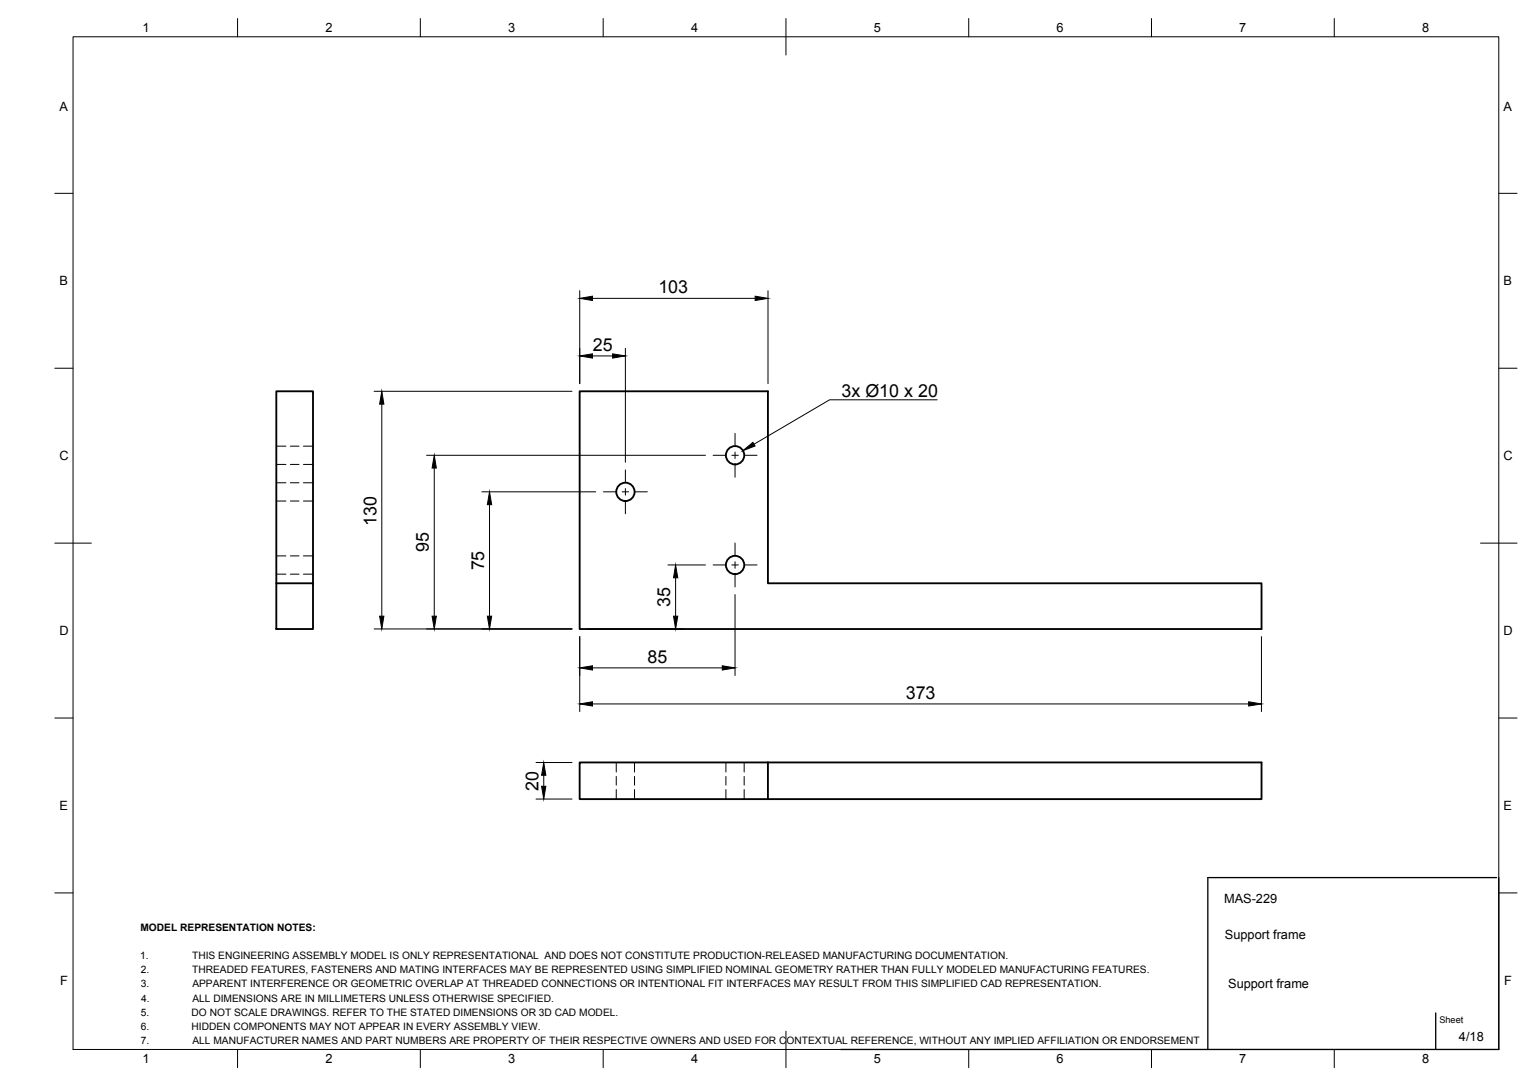
ISO-10303-21;
HEADER;
/* Generated by software containing ST-Developer
 * from STEP Tools, Inc. (www.steptools.com) 
 */

FILE_DESCRIPTION(
/* description */ ('Independently dimensioned six-bar single-leg walking-linkage demonstr
ator. Whole-mm20 crank,60 upper rocker,80/120 ternary coupler,120 lowe
r rocker,140 knee pitch and260 toe reach; ground pivots0/0,60/0,40/60.
 Seven native revolutes close both loops. Four reused native library f
amilies, fully retained shared pins and layered real spacer stacks, bo
nded rubber toe. Benchtop reference mechanism; no complete vehicle, lo
ad, gait stability, adhesive, weld, fit or life rating.'),
/* implementation_level */ '2;1');

FILE_NAME(
/* name */ 'Support frame.step',
/* time_stamp */ '2026-11-09T20:33:14-08:00',
/* author */ (''),
/* organization */ (''),
/* preprocessor_version */ 'ST-DEVELOPER v20.2',
/* originating_system */ 'Autodesk Translation Framework v15.17.0.0',
/* authorisation */ '');

FILE_SCHEMA (('AUTOMOTIVE_DESIGN { 1 0 10303 214 3 1 1 }'));
ENDSEC;

DATA;
#10=MECHANICAL_DESIGN_GEOMETRIC_PRESENTATION_REPRESENTATION('',(#256),#4048);
#220=SHAPE_REPRESENTATION_RELATIONSHIP('SRR','None',#4144,#238);
#238=ADVANCED_BREP_SHAPE_REPRESENTATION('',(#274),#4031);
#256=STYLED_ITEM('',(#4243),#274);
#274=MANIFOLD_SOLID_BREP('Body1',#2145);
#299=FACE_BOUND('',#569,.T.);
#300=FACE_BOUND('',#570,.T.);
#301=FACE_BOUND('',#571,.T.);
#302=FACE_BOUND('',#573,.T.);
#303=FACE_BOUND('',#574,.T.);
#304=FACE_BOUND('',#575,.T.);
#354=PLANE('',#2391);
#355=PLANE('',#2392);
#356=PLANE('',#2393);
#357=PLANE('',#2394);
#358=PLANE('',#2395);
#359=PLANE('',#2396);
#360=PLANE('',#2397);
#361=PLANE('',#2398);
#425=FACE_OUTER_BOUND('',#559,.T.);
#426=FACE_OUTER_BOUND('',#560,.T.);
#427=FACE_OUTER_BOUND('',#561,.T.);
#428=FACE_OUTER_BOUND('',#562,.T.);
#429=FACE_OUTER_BOUND('',#563,.T.);
#430=FACE_OUTER_BOUND('',#564,.T.);
#431=FACE_OUTER_BOUND('',#565,.T.);
#432=FACE_OUTER_BOUND('',#566,.T.);
#433=FACE_OUTER_BOUND('',#567,.T.);
#434=FACE_OUTER_BOUND('',#568,.T.);
#435=FACE_OUTER_BOUND('',#572,.T.);
#559=EDGE_LOOP('',(#1533,#1534,#1535,#1536));
#560=EDGE_LOOP('',(#1537,#1538,#1539,#1540));
#561=EDGE_LOOP('',(#1541,#1542,#1543,#1544));
#562=EDGE_LOOP('',(#1545,#1546,#1547,#1548));
#563=EDGE_LOOP('',(#1549,#1550,#1551,#1552));
#564=EDGE_LOOP('',(#1553,#1554,#1555,#1556));
#565=EDGE_LOOP('',(#1557,#1558,#1559,#1560));
#566=EDGE_LOOP('',(#1561,#1562,#1563,#1564));
#567=EDGE_LOOP('',(#1565,#1566,#1567,#1568));
#568=EDGE_LOOP('',(#1569,#1570,#1571,#1572,#1573,#1574));
#569=EDGE_LOOP('',(#1575));
#570=EDGE_LOOP('',(#1576));
#571=EDGE_LOOP('',(#1577));
#572=EDGE_LOOP('',(#1578,#1579,#1580,#1581,#1582,#1583));
#573=EDGE_LOOP('',(#1584));
#574=EDGE_LOOP('',(#1585));
#575=EDGE_LOOP('',(#1586));
#740=LINE('',#3473,#865);
#741=LINE('',#3479,#866);
#742=LINE('',#3485,#867);
#743=LINE('',#3490,#868);
#744=LINE('',#3492,#869);
#745=LINE('',#3494,#870);
#746=LINE('',#3495,#871);
#747=LINE('',#3498,#872);
#748=LINE('',#3500,#873);
#749=LINE('',#3501,#874);
#750=LINE('',#3504,#875);
#751=LINE('',#3506,#876);
#752=LINE('',#3507,#877);
#753=LINE('',#3511,#878);
#754=LINE('',#3513,#879);
#755=LINE('',#3515,#880);
#756=LINE('',#3516,#881);
#757=LINE('',#3518,#882);
#758=LINE('',#3519,#883);
#759=LINE('',#3521,#884);
#760=LINE('',#3522,#885);
#865=VECTOR('',#2733,5.);
#866=VECTOR('',#2740,5.);
#867=VECTOR('',#2747,5.);
#868=VECTOR('',#2752,10.);
#869=VECTOR('',#2753,10.);
#870=VECTOR('',#2754,10.);
#871=VECTOR('',#2755,10.);
#872=VECTOR('',#2758,10.);
#873=VECTOR('',#2759,10.);
#874=VECTOR('',#2760,10.);
#875=VECTOR('',#2763,10.);
#876=VECTOR('',#2764,10.);
#877=VECTOR('',#2765,10.);
#878=VECTOR('',#2768,10.);
#879=VECTOR('',#2769,10.);
#880=VECTOR('',#2770,10.);
#881=VECTOR('',#2771,10.);
#882=VECTOR('',#2774,10.);
#883=VECTOR('',#2775,10.);
#884=VECTOR('',#2778,10.);
#885=VECTOR('',#2779,10.);
#982=CIRCLE('',#2383,5.);
#983=CIRCLE('',#2384,5.);
#984=CIRCLE('',#2386,5.);
#985=CIRCLE('',#2387,5.);
#986=CIRCLE('',#2389,5.);
#987=CIRCLE('',#2390,5.);
#1104=VERTEX_POINT('',#3470);
#1105=VERTEX_POINT('',#3472);
#1106=VERTEX_POINT('',#3476);
#1107=VERTEX_POINT('',#3478);
#1108=VERTEX_POINT('',#3482);
#1109=VERTEX_POINT('',#3484);
#1110=VERTEX_POINT('',#3488);
#1111=VERTEX_POINT('',#3489);
#1112=VERTEX_POINT('',#3491);
#1113=VERTEX_POINT('',#3493);
#1114=VERTEX_POINT('',#3497);
#1115=VERTEX_POINT('',#3499);
#1116=VERTEX_POINT('',#3503);
#1117=VERTEX_POINT('',#3505);
#1118=VERTEX_POINT('',#3509);
#1119=VERTEX_POINT('',#3510);
#1120=VERTEX_POINT('',#3512);
#1121=VERTEX_POINT('',#3514);
#1270=EDGE_CURVE('',#1104,#1104,#982,.T.);
#1271=EDGE_CURVE('',#1104,#1105,#740,.T.);
#1272=EDGE_CURVE('',#1105,#1105,#983,.T.);
#1273=EDGE_CURVE('',#1106,#1106,#984,.T.);
#1274=EDGE_CURVE('',#1106,#1107,#741,.T.);
#1275=EDGE_CURVE('',#1107,#1107,#985,.T.);
#1276=EDGE_CURVE('',#1108,#1108,#986,.T.);
#1277=EDGE_CURVE('',#1108,#1109,#742,.T.);
#1278=EDGE_CURVE('',#1109,#1109,#987,.T.);
#1279=EDGE_CURVE('',#1110,#1111,#743,.T.);
#1280=EDGE_CURVE('',#1112,#1111,#744,.T.);
#1281=EDGE_CURVE('',#1113,#1112,#745,.T.);
#1282=EDGE_CURVE('',#1110,#1113,#746,.T.);
#1283=EDGE_CURVE('',#1114,#1110,#747,.T.);
#1284=EDGE_CURVE('',#1115,#1113,#748,.T.);
#1285=EDGE_CURVE('',#1114,#1115,#749,.T.);
#1286=EDGE_CURVE('',#1111,#1116,#750,.T.);
#1287=EDGE_CURVE('',#1116,#1117,#751,.F.);
#1288=EDGE_CURVE('',#1112,#1117,#752,.T.);
#1289=EDGE_CURVE('',#1118,#1119,#753,.F.);
#1290=EDGE_CURVE('',#1119,#1120,#754,.F.);
#1291=EDGE_CURVE('',#1121,#1120,#755,.F.);
#1292=EDGE_CURVE('',#1118,#1121,#756,.F.);
#1293=EDGE_CURVE('',#1116,#1118,#757,.F.);
#1294=EDGE_CURVE('',#1117,#1121,#758,.F.);
#1295=EDGE_CURVE('',#1119,#1114,#759,.F.);
#1296=EDGE_CURVE('',#1120,#1115,#760,.F.);
#1533=ORIENTED_EDGE('',*,*,#1270,.F.);
#1534=ORIENTED_EDGE('',*,*,#1271,.T.);
#1535=ORIENTED_EDGE('',*,*,#1272,.F.);
#1536=ORIENTED_EDGE('',*,*,#1271,.F.);
#1537=ORIENTED_EDGE('',*,*,#1273,.F.);
#1538=ORIENTED_EDGE('',*,*,#1274,.T.);
#1539=ORIENTED_EDGE('',*,*,#1275,.F.);
#1540=ORIENTED_EDGE('',*,*,#1274,.F.);
#1541=ORIENTED_EDGE('',*,*,#1276,.F.);
#1542=ORIENTED_EDGE('',*,*,#1277,.T.);
#1543=ORIENTED_EDGE('',*,*,#1278,.F.);
#1544=ORIENTED_EDGE('',*,*,#1277,.F.);
#1545=ORIENTED_EDGE('',*,*,#1279,.T.);
#1546=ORIENTED_EDGE('',*,*,#1280,.F.);
#1547=ORIENTED_EDGE('',*,*,#1281,.F.);
#1548=ORIENTED_EDGE('',*,*,#1282,.F.);
#1549=ORIENTED_EDGE('',*,*,#1283,.T.);
#1550=ORIENTED_EDGE('',*,*,#1282,.T.);
#1551=ORIENTED_EDGE('',*,*,#1284,.F.);
#1552=ORIENTED_EDGE('',*,*,#1285,.F.);
#1553=ORIENTED_EDGE('',*,*,#1280,.T.);
#1554=ORIENTED_EDGE('',*,*,#1286,.T.);
#1555=ORIENTED_EDGE('',*,*,#1287,.T.);
#1556=ORIENTED_EDGE('',*,*,#1288,.F.);
#1557=ORIENTED_EDGE('',*,*,#1289,.T.);
#1558=ORIENTED_EDGE('',*,*,#1290,.T.);
#1559=ORIENTED_EDGE('',*,*,#1291,.F.);
#1560=ORIENTED_EDGE('',*,*,#1292,.F.);
#1561=ORIENTED_EDGE('',*,*,#1293,.T.);
#1562=ORIENTED_EDGE('',*,*,#1292,.T.);
#1563=ORIENTED_EDGE('',*,*,#1294,.F.);
#1564=ORIENTED_EDGE('',*,*,#1287,.F.);
#1565=ORIENTED_EDGE('',*,*,#1295,.T.);
#1566=ORIENTED_EDGE('',*,*,#1285,.T.);
#1567=ORIENTED_EDGE('',*,*,#1296,.F.);
#1568=ORIENTED_EDGE('',*,*,#1290,.F.);
#1569=ORIENTED_EDGE('',*,*,#1296,.T.);
#1570=ORIENTED_EDGE('',*,*,#1284,.T.);
#1571=ORIENTED_EDGE('',*,*,#1281,.T.);
#1572=ORIENTED_EDGE('',*,*,#1288,.T.);
#1573=ORIENTED_EDGE('',*,*,#1294,.T.);
#1574=ORIENTED_EDGE('',*,*,#1291,.T.);
#1575=ORIENTED_EDGE('',*,*,#1270,.T.);
#1576=ORIENTED_EDGE('',*,*,#1273,.T.);
#1577=ORIENTED_EDGE('',*,*,#1276,.T.);
#1578=ORIENTED_EDGE('',*,*,#1295,.F.);
#1579=ORIENTED_EDGE('',*,*,#1289,.F.);
#1580=ORIENTED_EDGE('',*,*,#1293,.F.);
#1581=ORIENTED_EDGE('',*,*,#1286,.F.);
#1582=ORIENTED_EDGE('',*,*,#1279,.F.);
#1583=ORIENTED_EDGE('',*,*,#1283,.F.);
#1584=ORIENTED_EDGE('',*,*,#1272,.T.);
#1585=ORIENTED_EDGE('',*,*,#1275,.T.);
#1586=ORIENTED_EDGE('',*,*,#1278,.T.);
#1967=CYLINDRICAL_SURFACE('',#2382,5.);
#1968=CYLINDRICAL_SURFACE('',#2385,5.);
#1969=CYLINDRICAL_SURFACE('',#2388,5.);
#2028=ADVANCED_FACE('',(#425),#1967,.F.);
#2029=ADVANCED_FACE('',(#426),#1968,.F.);
#2030=ADVANCED_FACE('',(#427),#1969,.F.);
#2031=ADVANCED_FACE('',(#428),#354,.T.);
#2032=ADVANCED_FACE('',(#429),#355,.T.);
#2033=ADVANCED_FACE('',(#430),#356,.T.);
#2034=ADVANCED_FACE('',(#431),#357,.T.);
#2035=ADVANCED_FACE('',(#432),#358,.T.);
#2036=ADVANCED_FACE('',(#433),#359,.T.);
#2037=ADVANCED_FACE('',(#434,#299,#300,#301),#360,.T.);
#2038=ADVANCED_FACE('',(#435,#302,#303,#304),#361,.F.);
#2145=CLOSED_SHELL('',(#2028,#2029,#2030,#2031,#2032,#2033,#2034,#2035,
#2036,#2037,#2038));
#2381=AXIS2_PLACEMENT_3D('',#3468,#2727,#2728);
#2382=AXIS2_PLACEMENT_3D('',#3469,#2729,#2730);
#2383=AXIS2_PLACEMENT_3D('',#3471,#2731,#2732);
#2384=AXIS2_PLACEMENT_3D('',#3474,#2734,#2735);
#2385=AXIS2_PLACEMENT_3D('',#3475,#2736,#2737);
#2386=AXIS2_PLACEMENT_3D('',#3477,#2738,#2739);
#2387=AXIS2_PLACEMENT_3D('',#3480,#2741,#2742);
#2388=AXIS2_PLACEMENT_3D('',#3481,#2743,#2744);
#2389=AXIS2_PLACEMENT_3D('',#3483,#2745,#2746);
#2390=AXIS2_PLACEMENT_3D('',#3486,#2748,#2749);
#2391=AXIS2_PLACEMENT_3D('',#3487,#2750,#2751);
#2392=AXIS2_PLACEMENT_3D('',#3496,#2756,#2757);
#2393=AXIS2_PLACEMENT_3D('',#3502,#2761,#2762);
#2394=AXIS2_PLACEMENT_3D('',#3508,#2766,#2767);
#2395=AXIS2_PLACEMENT_3D('',#3517,#2772,#2773);
#2396=AXIS2_PLACEMENT_3D('',#3520,#2776,#2777);
#2397=AXIS2_PLACEMENT_3D('',#3523,#2780,#2781);
#2398=AXIS2_PLACEMENT_3D('',#3524,#2782,#2783);
#2727=DIRECTION('axis',(0.,0.,1.));
#2728=DIRECTION('refdir',(1.,0.,0.));
#2729=DIRECTION('center_axis',(0.,0.,-1.));
#2730=DIRECTION('ref_axis',(1.,0.,0.));
#2731=DIRECTION('center_axis',(0.,0.,-1.));
#2732=DIRECTION('ref_axis',(1.,0.,0.));
#2733=DIRECTION('',(0.,0.,-1.));
#2734=DIRECTION('center_axis',(0.,0.,1.));
#2735=DIRECTION('ref_axis',(1.,0.,0.));
#2736=DIRECTION('center_axis',(0.,0.,-1.));
#2737=DIRECTION('ref_axis',(1.,0.,0.));
#2738=DIRECTION('center_axis',(0.,0.,-1.));
#2739=DIRECTION('ref_axis',(1.,0.,0.));
#2740=DIRECTION('',(0.,0.,-1.));
#2741=DIRECTION('center_axis',(0.,0.,1.));
#2742=DIRECTION('ref_axis',(1.,0.,0.));
#2743=DIRECTION('center_axis',(0.,0.,-1.));
#2744=DIRECTION('ref_axis',(1.,0.,0.));
#2745=DIRECTION('center_axis',(0.,0.,-1.));
#2746=DIRECTION('ref_axis',(1.,0.,0.));
#2747=DIRECTION('',(0.,0.,-1.));
#2748=DIRECTION('center_axis',(0.,0.,1.));
#2749=DIRECTION('ref_axis',(1.,0.,0.));
#2750=DIRECTION('center_axis',(1.,0.,0.));
#2751=DIRECTION('ref_axis',(0.,1.,0.));
#2752=DIRECTION('',(0.,1.,0.));
#2753=DIRECTION('',(0.,0.,-1.));
#2754=DIRECTION('',(0.,1.,0.));
#2755=DIRECTION('',(0.,0.,1.));
#2756=DIRECTION('center_axis',(0.,-1.,0.));
#2757=DIRECTION('ref_axis',(1.,0.,0.));
#2758=DIRECTION('',(1.,0.,0.));
#2759=DIRECTION('',(1.,0.,0.));
#2760=DIRECTION('',(0.,0.,1.));
#2761=DIRECTION('center_axis',(0.,-1.,0.));
#2762=DIRECTION('ref_axis',(1.,0.,0.));
#2763=DIRECTION('',(1.,0.,0.));
#2764=DIRECTION('',(0.,0.,-1.));
#2765=DIRECTION('',(1.,0.,0.));
#2766=DIRECTION('center_axis',(0.,1.,0.));
#2767=DIRECTION('ref_axis',(-1.,0.,0.));
#2768=DIRECTION('',(1.,0.,0.));
#2769=DIRECTION('',(0.,0.,-1.));
#2770=DIRECTION('',(1.,0.,0.));
#2771=DIRECTION('',(0.,0.,-1.));
#2772=DIRECTION('center_axis',(1.,0.,0.));
#2773=DIRECTION('ref_axis',(0.,1.,0.));
#2774=DIRECTION('',(0.,-1.,0.));
#2775=DIRECTION('',(0.,-1.,0.));
#2776=DIRECTION('center_axis',(-1.,0.,0.));
#2777=DIRECTION('ref_axis',(0.,-1.,0.));
#2778=DIRECTION('',(0.,1.,0.));
#2779=DIRECTION('',(0.,1.,0.));
#2780=DIRECTION('center_axis',(0.,0.,1.));
#2781=DIRECTION('ref_axis',(1.,0.,0.));
#2782=DIRECTION('center_axis',(0.,0.,1.));
#2783=DIRECTION('ref_axis',(1.,0.,0.));
#3468=CARTESIAN_POINT('',(0.,0.,0.));
#3469=CARTESIAN_POINT('Origin',(60.,0.,10.));
#3470=CARTESIAN_POINT('',(55.,6.12323399573677E-16,20.));
#3471=CARTESIAN_POINT('Origin',(60.,0.,20.));
#3472=CARTESIAN_POINT('',(55.,6.12323399573677E-16,0.));
#3473=CARTESIAN_POINT('',(55.,6.12323399573677E-16,10.));
#3474=CARTESIAN_POINT('Origin',(60.,0.,0.));
#3475=CARTESIAN_POINT('Origin',(0.,0.,10.));
#3476=CARTESIAN_POINT('',(-5.,6.12323399573677E-16,20.));
#3477=CARTESIAN_POINT('Origin',(0.,0.,20.));
#3478=CARTESIAN_POINT('',(-5.,6.12323399573677E-16,0.));
#3479=CARTESIAN_POINT('',(-5.,6.12323399573677E-16,10.));
#3480=CARTESIAN_POINT('Origin',(0.,0.,0.));
#3481=CARTESIAN_POINT('Origin',(40.,60.,10.));
#3482=CARTESIAN_POINT('',(35.,60.,20.));
#3483=CARTESIAN_POINT('Origin',(40.,60.,20.));
#3484=CARTESIAN_POINT('',(35.,60.,0.));
#3485=CARTESIAN_POINT('',(35.,60.,10.));
#3486=CARTESIAN_POINT('Origin',(40.,60.,0.));
#3487=CARTESIAN_POINT('Origin',(-10.,-288.,0.));
#3488=CARTESIAN_POINT('',(-10.,-288.,0.));
#3489=CARTESIAN_POINT('',(-10.,-18.,0.));
#3490=CARTESIAN_POINT('',(-10.,-288.,0.));
#3491=CARTESIAN_POINT('',(-10.,-18.,20.));
#3492=CARTESIAN_POINT('',(-10.,-18.,0.));
#3493=CARTESIAN_POINT('',(-10.,-288.,20.));
#3494=CARTESIAN_POINT('',(-10.,-288.,20.));
#3495=CARTESIAN_POINT('',(-10.,-288.,0.));
#3496=CARTESIAN_POINT('Origin',(-30.,-288.,0.));
#3497=CARTESIAN_POINT('',(-35.,-288.,0.));
#3498=CARTESIAN_POINT('',(-30.,-288.,0.));
#3499=CARTESIAN_POINT('',(-35.,-288.,20.));
#3500=CARTESIAN_POINT('',(-30.,-288.,20.));
#3501=CARTESIAN_POINT('',(-35.,-288.,0.));
#3502=CARTESIAN_POINT('Origin',(-30.,-18.,0.));
#3503=CARTESIAN_POINT('',(95.,-18.,0.));
#3504=CARTESIAN_POINT('',(-30.,-18.,0.));
#3505=CARTESIAN_POINT('',(95.,-18.,20.));
#3506=CARTESIAN_POINT('',(95.,-18.,0.));
#3507=CARTESIAN_POINT('',(-30.,-18.,20.));
#3508=CARTESIAN_POINT('Origin',(90.,85.,0.));
#3509=CARTESIAN_POINT('',(95.,85.,0.));
#3510=CARTESIAN_POINT('',(-35.,85.,0.));
#3511=CARTESIAN_POINT('',(60.,85.,0.));
#3512=CARTESIAN_POINT('',(-35.,85.,20.));
#3513=CARTESIAN_POINT('',(-35.,85.,0.));
#3514=CARTESIAN_POINT('',(95.,85.,20.));
#3515=CARTESIAN_POINT('',(60.,85.,20.));
#3516=CARTESIAN_POINT('',(95.,85.,0.));
#3517=CARTESIAN_POINT('Origin',(95.,-18.,0.));
#3518=CARTESIAN_POINT('',(95.,6.5,0.));
#3519=CARTESIAN_POINT('',(95.,6.5,20.));
#3520=CARTESIAN_POINT('Origin',(-35.,80.,0.));
#3521=CARTESIAN_POINT('',(-35.,55.5,0.));
#3522=CARTESIAN_POINT('',(-35.,55.5,20.));
#3523=CARTESIAN_POINT('Origin',(30.,31.,20.));
#3524=CARTESIAN_POINT('Origin',(30.,31.,0.));
#4011=UNCERTAINTY_MEASURE_WITH_UNIT(LENGTH_MEASURE(0.01),#4049,
'DISTANCE_ACCURACY_VALUE',
'Maximum model space distance between geometric entities at asserted c
onnectivities');
#4028=UNCERTAINTY_MEASURE_WITH_UNIT(LENGTH_MEASURE(0.01),#4049,
'DISTANCE_ACCURACY_VALUE',
'Maximum model space distance between geometric entities at asserted c
onnectivities');
#4031=(
GEOMETRIC_REPRESENTATION_CONTEXT(3)
GLOBAL_UNCERTAINTY_ASSIGNED_CONTEXT((#4011))
GLOBAL_UNIT_ASSIGNED_CONTEXT((#4049,#4051,#4052))
REPRESENTATION_CONTEXT('','3D')
);
#4048=(
GEOMETRIC_REPRESENTATION_CONTEXT(3)
GLOBAL_UNCERTAINTY_ASSIGNED_CONTEXT((#4028))
GLOBAL_UNIT_ASSIGNED_CONTEXT((#4049,#4051,#4052))
REPRESENTATION_CONTEXT('','3D')
);
#4049=(
LENGTH_UNIT()
NAMED_UNIT(*)
SI_UNIT(.MILLI.,.METRE.)
);
#4051=(
NAMED_UNIT(*)
PLANE_ANGLE_UNIT()
SI_UNIT($,.RADIAN.)
);
#4052=(
NAMED_UNIT(*)
SI_UNIT($,.STERADIAN.)
SOLID_ANGLE_UNIT()
);
#4055=SHAPE_DEFINITION_REPRESENTATION(#4074,#4144);
#4074=PRODUCT_DEFINITION_SHAPE('',$,#4164);
#4144=SHAPE_REPRESENTATION('',(#2381),#4031);
#4161=PRODUCT_DEFINITION_CONTEXT('part definition',#4220,'design');
#4164=PRODUCT_DEFINITION('Support frame','Support frame',#4183,#4161);
#4183=PRODUCT_DEFINITION_FORMATION('',$,#4224);
#4220=APPLICATION_CONTEXT(
'Core Data for Automotive Mechanical Design Process');
#4221=PRODUCT_CONTEXT('part definition',#4220,'mechanical');
#4224=PRODUCT('Support frame','Support frame','Support frame',(#4221));
#4243=PRESENTATION_STYLE_ASSIGNMENT((#4257));
#4257=SURFACE_STYLE_USAGE(.BOTH.,#4271);
#4271=SURFACE_SIDE_STYLE('',(#4285));
#4285=SURFACE_STYLE_FILL_AREA(#4299);
#4299=FILL_AREA_STYLE('Frame gray',(#4313));
#4313=FILL_AREA_STYLE_COLOUR('Frame gray',#4327);
#4327=COLOUR_RGB('Frame gray',0.407843137254902,0.447058823529412,0.498039215686275);
ENDSEC;
END-ISO-10303-21;
